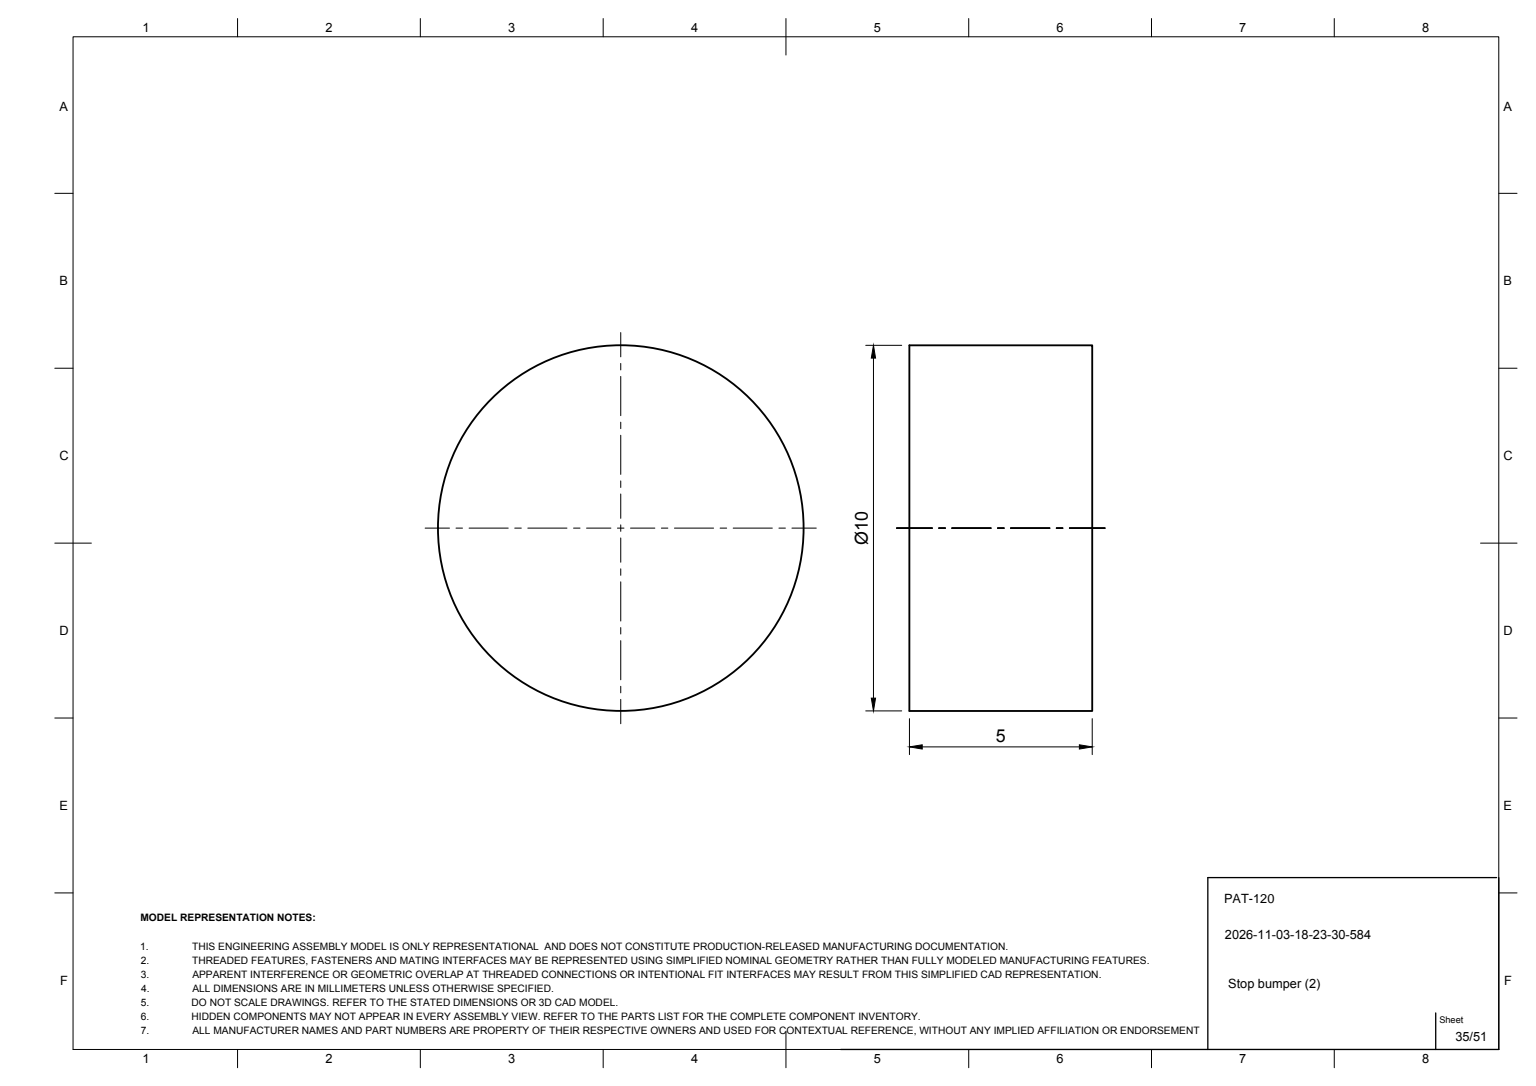
ISO-10303-21;
HEADER;
/* Generated by software containing ST-Developer
 * from STEP Tools, Inc. (www.steptools.com) 
 */

FILE_DESCRIPTION(
/* description */ ('Vibration shaker table dummy'),
/* implementation_level */ '2;1');

FILE_NAME(
/* name */ 'Stop bumper (2).step',
/* time_stamp */ '2026-10-27T10:55:14-07:00',
/* author */ (''),
/* organization */ (''),
/* preprocessor_version */ 'ST-DEVELOPER v20.2',
/* originating_system */ 'Autodesk Translation Framework v15.17.0.0',
/* authorisation */ '');

FILE_SCHEMA (('AUTOMOTIVE_DESIGN { 1 0 10303 214 3 1 1 }'));
ENDSEC;

DATA;
#10=MECHANICAL_DESIGN_GEOMETRIC_PRESENTATION_REPRESENTATION('',(#716),#22394);
#624=SHAPE_REPRESENTATION_RELATIONSHIP('SRR','None',#22670,#670);
#670=ADVANCED_BREP_SHAPE_REPRESENTATION('',(#762),#22376);
#716=STYLED_ITEM('',(#22975),#762);
#762=MANIFOLD_SOLID_BREP('Body1',#9234);
#1225=PLANE('',#10321);
#1226=PLANE('',#10322);
#1622=FACE_OUTER_BOUND('',#2291,.T.);
#1623=FACE_OUTER_BOUND('',#2292,.T.);
#1624=FACE_OUTER_BOUND('',#2293,.T.);
#2291=EDGE_LOOP('',(#7470,#7471,#7472,#7473));
#2292=EDGE_LOOP('',(#7474));
#2293=EDGE_LOOP('',(#7475));
#2982=LINE('',#21065,#3601);
#3601=VECTOR('',#12430,0.5);
#4108=CIRCLE('',#10319,0.5);
#4109=CIRCLE('',#10320,0.5);
#4775=VERTEX_POINT('',#21062);
#4776=VERTEX_POINT('',#21064);
#5728=EDGE_CURVE('',#4775,#4775,#4108,.T.);
#5729=EDGE_CURVE('',#4775,#4776,#2982,.T.);
#5730=EDGE_CURVE('',#4776,#4776,#4109,.T.);
#7470=ORIENTED_EDGE('',*,*,#5728,.F.);
#7471=ORIENTED_EDGE('',*,*,#5729,.T.);
#7472=ORIENTED_EDGE('',*,*,#5730,.T.);
#7473=ORIENTED_EDGE('',*,*,#5729,.F.);
#7474=ORIENTED_EDGE('',*,*,#5728,.T.);
#7475=ORIENTED_EDGE('',*,*,#5730,.F.);
#8618=CYLINDRICAL_SURFACE('',#10318,0.5);
#8987=ADVANCED_FACE('',(#1622),#8618,.T.);
#8988=ADVANCED_FACE('',(#1623),#1225,.T.);
#8989=ADVANCED_FACE('',(#1624),#1226,.F.);
#9234=CLOSED_SHELL('',(#8987,#8988,#8989));
#10317=AXIS2_PLACEMENT_3D('',#21060,#12424,#12425);
#10318=AXIS2_PLACEMENT_3D('',#21061,#12426,#12427);
#10319=AXIS2_PLACEMENT_3D('',#21063,#12428,#12429);
#10320=AXIS2_PLACEMENT_3D('',#21066,#12431,#12432);
#10321=AXIS2_PLACEMENT_3D('',#21067,#12433,#12434);
#10322=AXIS2_PLACEMENT_3D('',#21068,#12435,#12436);
#12424=DIRECTION('axis',(0.,0.,1.));
#12425=DIRECTION('refdir',(1.,0.,0.));
#12426=DIRECTION('center_axis',(0.,0.,1.));
#12427=DIRECTION('ref_axis',(1.,0.,0.));
#12428=DIRECTION('center_axis',(0.,0.,1.));
#12429=DIRECTION('ref_axis',(1.,0.,0.));
#12430=DIRECTION('',(0.,0.,-1.));
#12431=DIRECTION('center_axis',(0.,0.,1.));
#12432=DIRECTION('ref_axis',(1.,0.,0.));
#12433=DIRECTION('center_axis',(0.,0.,1.));
#12434=DIRECTION('ref_axis',(1.,0.,0.));
#12435=DIRECTION('center_axis',(0.,0.,1.));
#12436=DIRECTION('ref_axis',(1.,0.,0.));
#21060=CARTESIAN_POINT('',(0.,0.,0.));
#21061=CARTESIAN_POINT('Origin',(0.,6.,13.6));
#21062=CARTESIAN_POINT('',(-0.5,6.,14.1));
#21063=CARTESIAN_POINT('Origin',(0.,6.,14.1));
#21064=CARTESIAN_POINT('',(-0.5,6.,13.6));
#21065=CARTESIAN_POINT('',(-0.5,6.,13.6));
#21066=CARTESIAN_POINT('Origin',(0.,6.,13.6));
#21067=CARTESIAN_POINT('Origin',(0.,6.,14.1));
#21068=CARTESIAN_POINT('Origin',(0.,6.,13.6));
#22325=UNCERTAINTY_MEASURE_WITH_UNIT(LENGTH_MEASURE(0.001),#22395,
'DISTANCE_ACCURACY_VALUE',
'Maximum model space distance between geometric entities at asserted c
onnectivities');
#22343=UNCERTAINTY_MEASURE_WITH_UNIT(LENGTH_MEASURE(0.001),#22395,
'DISTANCE_ACCURACY_VALUE',
'Maximum model space distance between geometric entities at asserted c
onnectivities');
#22376=(
GEOMETRIC_REPRESENTATION_CONTEXT(3)
GLOBAL_UNCERTAINTY_ASSIGNED_CONTEXT((#22325))
GLOBAL_UNIT_ASSIGNED_CONTEXT((#22395,#22397,#22398))
REPRESENTATION_CONTEXT('','3D')
);
#22394=(
GEOMETRIC_REPRESENTATION_CONTEXT(3)
GLOBAL_UNCERTAINTY_ASSIGNED_CONTEXT((#22343))
GLOBAL_UNIT_ASSIGNED_CONTEXT((#22395,#22397,#22398))
REPRESENTATION_CONTEXT('','3D')
);
#22395=(
LENGTH_UNIT()
NAMED_UNIT(*)
SI_UNIT(.CENTI.,.METRE.)
);
#22397=(
NAMED_UNIT(*)
PLANE_ANGLE_UNIT()
SI_UNIT($,.RADIAN.)
);
#22398=(
NAMED_UNIT(*)
SI_UNIT($,.STERADIAN.)
SOLID_ANGLE_UNIT()
);
#22431=SHAPE_DEFINITION_REPRESENTATION(#22481,#22670);
#22481=PRODUCT_DEFINITION_SHAPE('',$,#22721);
#22670=SHAPE_REPRESENTATION('',(#10317),#22376);
#22688=PRODUCT_DEFINITION_CONTEXT('part definition',#22840,'design');
#22721=PRODUCT_DEFINITION('Stop bumper (2)','Stop bumper (2)',#22771,#22688);
#22771=PRODUCT_DEFINITION_FORMATION('',$,#22874);
#22840=APPLICATION_CONTEXT(
'Core Data for Automotive Mechanical Design Process');
#22841=PRODUCT_CONTEXT('part definition',#22840,'mechanical');
#22874=PRODUCT('Stop bumper (2)','Stop bumper (2)','Stop bumper (2)',(#22841));
#22969=COLOUR_RGB('Off White',0.89,0.88,0.83);
#22970=FILL_AREA_STYLE_COLOUR('',#22969);
#22971=FILL_AREA_STYLE('',(#22970));
#22972=SURFACE_STYLE_FILL_AREA(#22971);
#22973=SURFACE_SIDE_STYLE('',(#22972));
#22974=SURFACE_STYLE_USAGE(.BOTH.,#22973);
#22975=PRESENTATION_STYLE_ASSIGNMENT((#22974));
ENDSEC;
END-ISO-10303-21;
